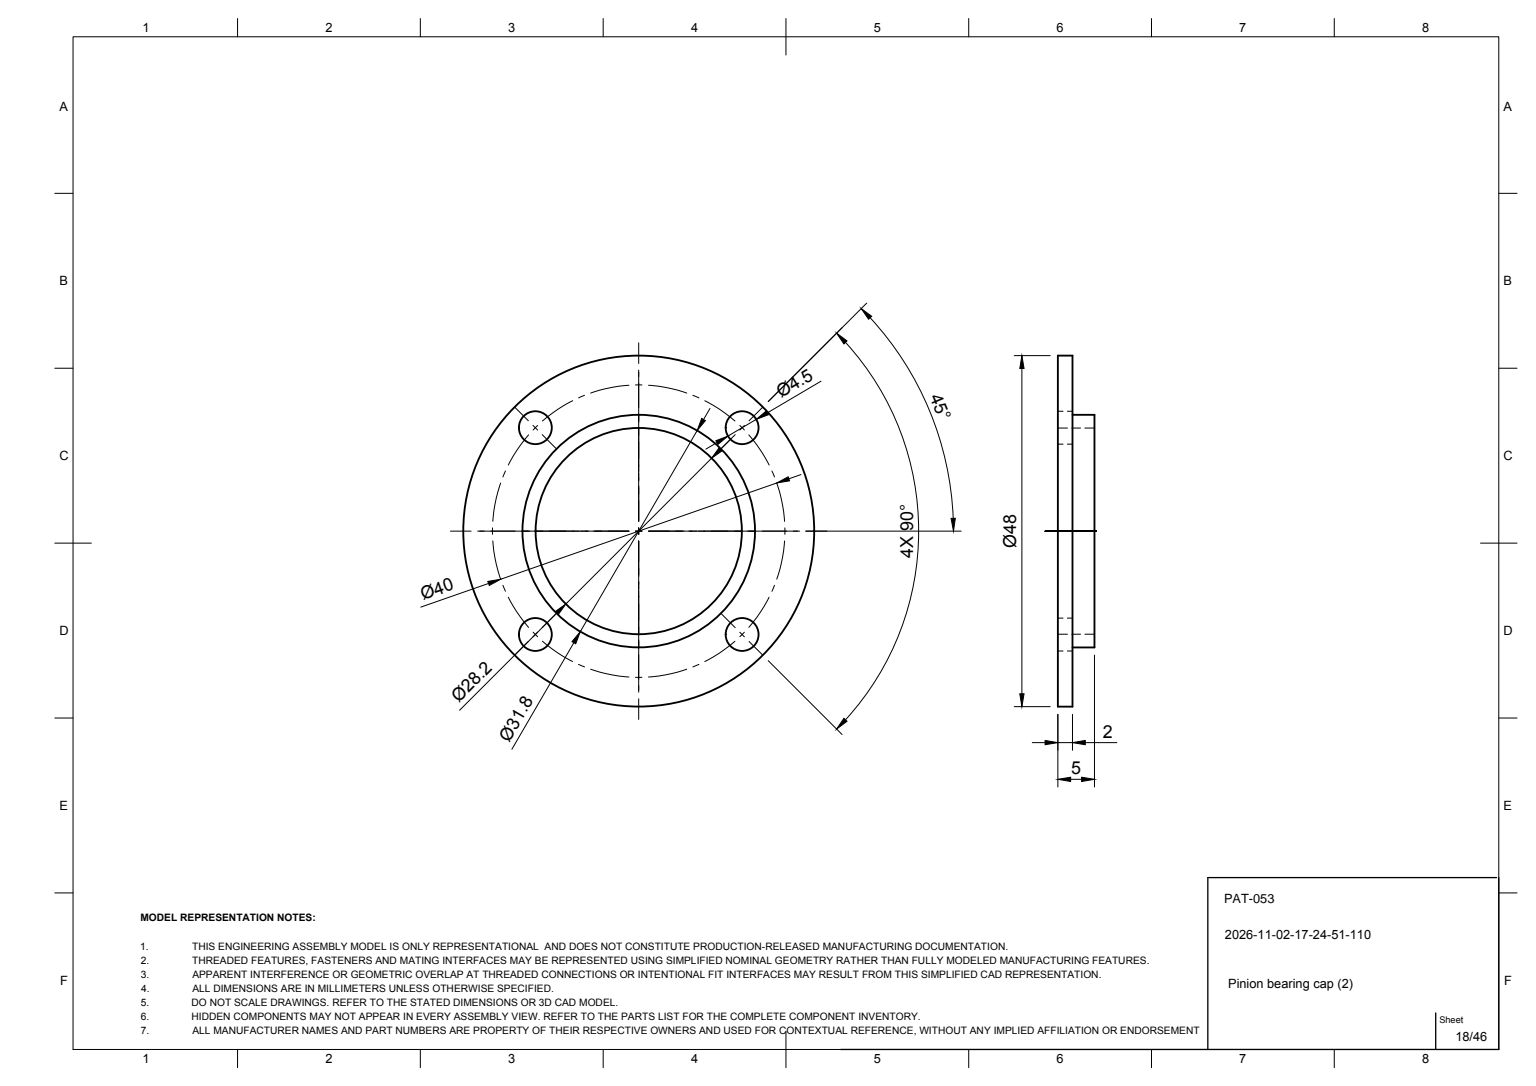
ISO-10303-21;
HEADER;
/* Generated by software containing ST-Developer
 * from STEP Tools, Inc. (www.steptools.com) 
 */

FILE_DESCRIPTION(
/* description */ ('Hand-operated arbor press'),
/* implementation_level */ '2;1');

FILE_NAME(
/* name */ 'Pinion bearing cap (2).step',
/* time_stamp */ '2026-10-28T03:25:25-07:00',
/* author */ (''),
/* organization */ (''),
/* preprocessor_version */ 'ST-DEVELOPER v20.2',
/* originating_system */ 'Autodesk Translation Framework v15.17.0.0',
/* authorisation */ '');

FILE_SCHEMA (('AUTOMOTIVE_DESIGN { 1 0 10303 214 3 1 1 }'));
ENDSEC;

DATA;
#10=MECHANICAL_DESIGN_GEOMETRIC_PRESENTATION_REPRESENTATION('',(#599),#32751);
#515=SHAPE_REPRESENTATION_RELATIONSHIP('SRR','None',#32944,#557);
#557=ADVANCED_BREP_SHAPE_REPRESENTATION('',(#648),#32718);
#599=STYLED_ITEM('',(#33242),#648);
#648=MANIFOLD_SOLID_BREP('Body1',#12496);
#779=FACE_BOUND('',#2262,.T.);
#780=FACE_BOUND('',#2265,.T.);
#781=FACE_BOUND('',#2266,.T.);
#782=FACE_BOUND('',#2267,.T.);
#783=FACE_BOUND('',#2268,.T.);
#784=FACE_BOUND('',#2269,.T.);
#785=FACE_BOUND('',#2271,.T.);
#786=FACE_BOUND('',#2272,.T.);
#787=FACE_BOUND('',#2273,.T.);
#788=FACE_BOUND('',#2274,.T.);
#789=FACE_BOUND('',#2275,.T.);
#960=PLANE('',#13357);
#961=PLANE('',#13361);
#962=PLANE('',#13362);
#1475=FACE_OUTER_BOUND('',#2255,.T.);
#1476=FACE_OUTER_BOUND('',#2256,.T.);
#1477=FACE_OUTER_BOUND('',#2257,.T.);
#1478=FACE_OUTER_BOUND('',#2258,.T.);
#1479=FACE_OUTER_BOUND('',#2259,.T.);
#1480=FACE_OUTER_BOUND('',#2260,.T.);
#1481=FACE_OUTER_BOUND('',#2261,.T.);
#1482=FACE_OUTER_BOUND('',#2263,.T.);
#1483=FACE_OUTER_BOUND('',#2264,.T.);
#1484=FACE_OUTER_BOUND('',#2270,.T.);
#2255=EDGE_LOOP('',(#9194,#9195,#9196,#9197));
#2256=EDGE_LOOP('',(#9198,#9199,#9200,#9201));
#2257=EDGE_LOOP('',(#9202,#9203,#9204,#9205));
#2258=EDGE_LOOP('',(#9206,#9207,#9208,#9209));
#2259=EDGE_LOOP('',(#9210,#9211,#9212,#9213));
#2260=EDGE_LOOP('',(#9214,#9215,#9216,#9217));
#2261=EDGE_LOOP('',(#9218));
#2262=EDGE_LOOP('',(#9219));
#2263=EDGE_LOOP('',(#9220,#9221,#9222,#9223));
#2264=EDGE_LOOP('',(#9224));
#2265=EDGE_LOOP('',(#9225));
#2266=EDGE_LOOP('',(#9226));
#2267=EDGE_LOOP('',(#9227));
#2268=EDGE_LOOP('',(#9228));
#2269=EDGE_LOOP('',(#9229));
#2270=EDGE_LOOP('',(#9230));
#2271=EDGE_LOOP('',(#9231));
#2272=EDGE_LOOP('',(#9232));
#2273=EDGE_LOOP('',(#9233));
#2274=EDGE_LOOP('',(#9234));
#2275=EDGE_LOOP('',(#9235));
#3117=LINE('',#18565,#4288);
#3118=LINE('',#18571,#4289);
#3119=LINE('',#18577,#4290);
#3120=LINE('',#18583,#4291);
#3121=LINE('',#18589,#4292);
#3122=LINE('',#18595,#4293);
#3123=LINE('',#18602,#4294);
#4288=VECTOR('',#15132,1.41);
#4289=VECTOR('',#15139,0.225);
#4290=VECTOR('',#15146,0.225);
#4291=VECTOR('',#15153,0.225);
#4292=VECTOR('',#15160,0.225);
#4293=VECTOR('',#15167,1.59);
#4294=VECTOR('',#15176,2.4);
#5308=CIRCLE('',#13340,1.41);
#5309=CIRCLE('',#13341,1.41);
#5310=CIRCLE('',#13343,0.225);
#5311=CIRCLE('',#13344,0.225);
#5312=CIRCLE('',#13346,0.225);
#5313=CIRCLE('',#13347,0.225);
#5314=CIRCLE('',#13349,0.225);
#5315=CIRCLE('',#13350,0.225);
#5316=CIRCLE('',#13352,0.225);
#5317=CIRCLE('',#13353,0.225);
#5318=CIRCLE('',#13355,1.59);
#5319=CIRCLE('',#13356,1.59);
#5320=CIRCLE('',#13359,2.4);
#5321=CIRCLE('',#13360,2.4);
#5846=VERTEX_POINT('',#18562);
#5847=VERTEX_POINT('',#18564);
#5848=VERTEX_POINT('',#18568);
#5849=VERTEX_POINT('',#18570);
#5850=VERTEX_POINT('',#18574);
#5851=VERTEX_POINT('',#18576);
#5852=VERTEX_POINT('',#18580);
#5853=VERTEX_POINT('',#18582);
#5854=VERTEX_POINT('',#18586);
#5855=VERTEX_POINT('',#18588);
#5856=VERTEX_POINT('',#18592);
#5857=VERTEX_POINT('',#18594);
#5858=VERTEX_POINT('',#18599);
#5859=VERTEX_POINT('',#18601);
#7100=EDGE_CURVE('',#5846,#5846,#5308,.T.);
#7101=EDGE_CURVE('',#5846,#5847,#3117,.T.);
#7102=EDGE_CURVE('',#5847,#5847,#5309,.T.);
#7103=EDGE_CURVE('',#5848,#5848,#5310,.T.);
#7104=EDGE_CURVE('',#5848,#5849,#3118,.T.);
#7105=EDGE_CURVE('',#5849,#5849,#5311,.T.);
#7106=EDGE_CURVE('',#5850,#5850,#5312,.T.);
#7107=EDGE_CURVE('',#5850,#5851,#3119,.T.);
#7108=EDGE_CURVE('',#5851,#5851,#5313,.T.);
#7109=EDGE_CURVE('',#5852,#5852,#5314,.T.);
#7110=EDGE_CURVE('',#5852,#5853,#3120,.T.);
#7111=EDGE_CURVE('',#5853,#5853,#5315,.T.);
#7112=EDGE_CURVE('',#5854,#5854,#5316,.T.);
#7113=EDGE_CURVE('',#5854,#5855,#3121,.T.);
#7114=EDGE_CURVE('',#5855,#5855,#5317,.T.);
#7115=EDGE_CURVE('',#5856,#5856,#5318,.T.);
#7116=EDGE_CURVE('',#5856,#5857,#3122,.T.);
#7117=EDGE_CURVE('',#5857,#5857,#5319,.T.);
#7118=EDGE_CURVE('',#5858,#5858,#5320,.T.);
#7119=EDGE_CURVE('',#5858,#5859,#3123,.T.);
#7120=EDGE_CURVE('',#5859,#5859,#5321,.T.);
#9194=ORIENTED_EDGE('',*,*,#7100,.F.);
#9195=ORIENTED_EDGE('',*,*,#7101,.T.);
#9196=ORIENTED_EDGE('',*,*,#7102,.F.);
#9197=ORIENTED_EDGE('',*,*,#7101,.F.);
#9198=ORIENTED_EDGE('',*,*,#7103,.F.);
#9199=ORIENTED_EDGE('',*,*,#7104,.T.);
#9200=ORIENTED_EDGE('',*,*,#7105,.F.);
#9201=ORIENTED_EDGE('',*,*,#7104,.F.);
#9202=ORIENTED_EDGE('',*,*,#7106,.F.);
#9203=ORIENTED_EDGE('',*,*,#7107,.T.);
#9204=ORIENTED_EDGE('',*,*,#7108,.F.);
#9205=ORIENTED_EDGE('',*,*,#7107,.F.);
#9206=ORIENTED_EDGE('',*,*,#7109,.F.);
#9207=ORIENTED_EDGE('',*,*,#7110,.T.);
#9208=ORIENTED_EDGE('',*,*,#7111,.F.);
#9209=ORIENTED_EDGE('',*,*,#7110,.F.);
#9210=ORIENTED_EDGE('',*,*,#7112,.F.);
#9211=ORIENTED_EDGE('',*,*,#7113,.T.);
#9212=ORIENTED_EDGE('',*,*,#7114,.F.);
#9213=ORIENTED_EDGE('',*,*,#7113,.F.);
#9214=ORIENTED_EDGE('',*,*,#7115,.F.);
#9215=ORIENTED_EDGE('',*,*,#7116,.T.);
#9216=ORIENTED_EDGE('',*,*,#7117,.F.);
#9217=ORIENTED_EDGE('',*,*,#7116,.F.);
#9218=ORIENTED_EDGE('',*,*,#7115,.T.);
#9219=ORIENTED_EDGE('',*,*,#7102,.T.);
#9220=ORIENTED_EDGE('',*,*,#7118,.F.);
#9221=ORIENTED_EDGE('',*,*,#7119,.T.);
#9222=ORIENTED_EDGE('',*,*,#7120,.T.);
#9223=ORIENTED_EDGE('',*,*,#7119,.F.);
#9224=ORIENTED_EDGE('',*,*,#7118,.T.);
#9225=ORIENTED_EDGE('',*,*,#7117,.T.);
#9226=ORIENTED_EDGE('',*,*,#7114,.T.);
#9227=ORIENTED_EDGE('',*,*,#7111,.T.);
#9228=ORIENTED_EDGE('',*,*,#7108,.T.);
#9229=ORIENTED_EDGE('',*,*,#7105,.T.);
#9230=ORIENTED_EDGE('',*,*,#7120,.F.);
#9231=ORIENTED_EDGE('',*,*,#7100,.T.);
#9232=ORIENTED_EDGE('',*,*,#7112,.T.);
#9233=ORIENTED_EDGE('',*,*,#7109,.T.);
#9234=ORIENTED_EDGE('',*,*,#7106,.T.);
#9235=ORIENTED_EDGE('',*,*,#7103,.T.);
#11713=CYLINDRICAL_SURFACE('',#13339,1.41);
#11714=CYLINDRICAL_SURFACE('',#13342,0.225);
#11715=CYLINDRICAL_SURFACE('',#13345,0.225);
#11716=CYLINDRICAL_SURFACE('',#13348,0.225);
#11717=CYLINDRICAL_SURFACE('',#13351,0.225);
#11718=CYLINDRICAL_SURFACE('',#13354,1.59);
#11719=CYLINDRICAL_SURFACE('',#13358,2.4);
#11984=ADVANCED_FACE('',(#1475),#11713,.F.);
#11985=ADVANCED_FACE('',(#1476),#11714,.F.);
#11986=ADVANCED_FACE('',(#1477),#11715,.F.);
#11987=ADVANCED_FACE('',(#1478),#11716,.F.);
#11988=ADVANCED_FACE('',(#1479),#11717,.F.);
#11989=ADVANCED_FACE('',(#1480),#11718,.T.);
#11990=ADVANCED_FACE('',(#1481,#779),#960,.T.);
#11991=ADVANCED_FACE('',(#1482),#11719,.T.);
#11992=ADVANCED_FACE('',(#1483,#780,#781,#782,#783,#784),#961,.T.);
#11993=ADVANCED_FACE('',(#1484,#785,#786,#787,#788,#789),#962,.F.);
#12496=CLOSED_SHELL('',(#11984,#11985,#11986,#11987,#11988,#11989,#11990,
#11991,#11992,#11993));
#13338=AXIS2_PLACEMENT_3D('',#18560,#15126,#15127);
#13339=AXIS2_PLACEMENT_3D('',#18561,#15128,#15129);
#13340=AXIS2_PLACEMENT_3D('',#18563,#15130,#15131);
#13341=AXIS2_PLACEMENT_3D('',#18566,#15133,#15134);
#13342=AXIS2_PLACEMENT_3D('',#18567,#15135,#15136);
#13343=AXIS2_PLACEMENT_3D('',#18569,#15137,#15138);
#13344=AXIS2_PLACEMENT_3D('',#18572,#15140,#15141);
#13345=AXIS2_PLACEMENT_3D('',#18573,#15142,#15143);
#13346=AXIS2_PLACEMENT_3D('',#18575,#15144,#15145);
#13347=AXIS2_PLACEMENT_3D('',#18578,#15147,#15148);
#13348=AXIS2_PLACEMENT_3D('',#18579,#15149,#15150);
#13349=AXIS2_PLACEMENT_3D('',#18581,#15151,#15152);
#13350=AXIS2_PLACEMENT_3D('',#18584,#15154,#15155);
#13351=AXIS2_PLACEMENT_3D('',#18585,#15156,#15157);
#13352=AXIS2_PLACEMENT_3D('',#18587,#15158,#15159);
#13353=AXIS2_PLACEMENT_3D('',#18590,#15161,#15162);
#13354=AXIS2_PLACEMENT_3D('',#18591,#15163,#15164);
#13355=AXIS2_PLACEMENT_3D('',#18593,#15165,#15166);
#13356=AXIS2_PLACEMENT_3D('',#18596,#15168,#15169);
#13357=AXIS2_PLACEMENT_3D('',#18597,#15170,#15171);
#13358=AXIS2_PLACEMENT_3D('',#18598,#15172,#15173);
#13359=AXIS2_PLACEMENT_3D('',#18600,#15174,#15175);
#13360=AXIS2_PLACEMENT_3D('',#18603,#15177,#15178);
#13361=AXIS2_PLACEMENT_3D('',#18604,#15179,#15180);
#13362=AXIS2_PLACEMENT_3D('',#18605,#15181,#15182);
#15126=DIRECTION('axis',(0.,0.,1.));
#15127=DIRECTION('refdir',(1.,0.,0.));
#15128=DIRECTION('center_axis',(0.,1.,0.));
#15129=DIRECTION('ref_axis',(1.,0.,0.));
#15130=DIRECTION('center_axis',(0.,1.,0.));
#15131=DIRECTION('ref_axis',(1.,0.,0.));
#15132=DIRECTION('',(0.,1.,0.));
#15133=DIRECTION('center_axis',(0.,-1.,0.));
#15134=DIRECTION('ref_axis',(1.,0.,0.));
#15135=DIRECTION('center_axis',(0.,1.,0.));
#15136=DIRECTION('ref_axis',(1.,0.,0.));
#15137=DIRECTION('center_axis',(0.,1.,0.));
#15138=DIRECTION('ref_axis',(1.,0.,0.));
#15139=DIRECTION('',(0.,1.,0.));
#15140=DIRECTION('center_axis',(0.,-1.,0.));
#15141=DIRECTION('ref_axis',(1.,0.,0.));
#15142=DIRECTION('center_axis',(0.,1.,0.));
#15143=DIRECTION('ref_axis',(1.,0.,0.));
#15144=DIRECTION('center_axis',(0.,1.,0.));
#15145=DIRECTION('ref_axis',(1.,0.,0.));
#15146=DIRECTION('',(0.,1.,0.));
#15147=DIRECTION('center_axis',(0.,-1.,0.));
#15148=DIRECTION('ref_axis',(1.,0.,0.));
#15149=DIRECTION('center_axis',(0.,1.,0.));
#15150=DIRECTION('ref_axis',(1.,0.,0.));
#15151=DIRECTION('center_axis',(0.,1.,0.));
#15152=DIRECTION('ref_axis',(1.,0.,0.));
#15153=DIRECTION('',(0.,1.,0.));
#15154=DIRECTION('center_axis',(0.,-1.,0.));
#15155=DIRECTION('ref_axis',(1.,0.,0.));
#15156=DIRECTION('center_axis',(0.,1.,0.));
#15157=DIRECTION('ref_axis',(1.,0.,0.));
#15158=DIRECTION('center_axis',(0.,1.,0.));
#15159=DIRECTION('ref_axis',(1.,0.,0.));
#15160=DIRECTION('',(0.,1.,0.));
#15161=DIRECTION('center_axis',(0.,-1.,0.));
#15162=DIRECTION('ref_axis',(1.,0.,0.));
#15163=DIRECTION('center_axis',(0.,1.,0.));
#15164=DIRECTION('ref_axis',(1.,0.,0.));
#15165=DIRECTION('center_axis',(0.,1.,0.));
#15166=DIRECTION('ref_axis',(1.,0.,0.));
#15167=DIRECTION('',(0.,-1.,0.));
#15168=DIRECTION('center_axis',(0.,-1.,0.));
#15169=DIRECTION('ref_axis',(1.,0.,0.));
#15170=DIRECTION('center_axis',(0.,1.,0.));
#15171=DIRECTION('ref_axis',(1.,0.,0.));
#15172=DIRECTION('center_axis',(0.,1.,0.));
#15173=DIRECTION('ref_axis',(1.,0.,0.));
#15174=DIRECTION('center_axis',(0.,1.,0.));
#15175=DIRECTION('ref_axis',(1.,0.,0.));
#15176=DIRECTION('',(0.,-1.,0.));
#15177=DIRECTION('center_axis',(0.,1.,0.));
#15178=DIRECTION('ref_axis',(1.,0.,0.));
#15179=DIRECTION('center_axis',(0.,1.,0.));
#15180=DIRECTION('ref_axis',(1.,0.,0.));
#15181=DIRECTION('center_axis',(0.,1.,0.));
#15182=DIRECTION('ref_axis',(1.,0.,0.));
#18560=CARTESIAN_POINT('',(0.,0.,0.));
#18561=CARTESIAN_POINT('Origin',(-3.25,-4.1,20.));
#18562=CARTESIAN_POINT('',(-4.66,2.,20.));
#18563=CARTESIAN_POINT('Origin',(-3.25,2.,20.));
#18564=CARTESIAN_POINT('',(-4.66,2.5,20.));
#18565=CARTESIAN_POINT('',(-4.66,-4.1,20.));
#18566=CARTESIAN_POINT('Origin',(-3.25,2.5,20.));
#18567=CARTESIAN_POINT('Origin',(-4.66421356237309,1.9,18.5857864376269));
#18568=CARTESIAN_POINT('',(-4.88921356237309,2.,18.5857864376269));
#18569=CARTESIAN_POINT('Origin',(-4.66421356237309,2.,18.5857864376269));
#18570=CARTESIAN_POINT('',(-4.88921356237309,2.2,18.5857864376269));
#18571=CARTESIAN_POINT('',(-4.88921356237309,1.9,18.5857864376269));
#18572=CARTESIAN_POINT('Origin',(-4.66421356237309,2.2,18.5857864376269));
#18573=CARTESIAN_POINT('Origin',(-4.66421356237309,1.9,21.4142135623731));
#18574=CARTESIAN_POINT('',(-4.88921356237309,2.,21.4142135623731));
#18575=CARTESIAN_POINT('Origin',(-4.66421356237309,2.,21.4142135623731));
#18576=CARTESIAN_POINT('',(-4.88921356237309,2.2,21.4142135623731));
#18577=CARTESIAN_POINT('',(-4.88921356237309,1.9,21.4142135623731));
#18578=CARTESIAN_POINT('Origin',(-4.66421356237309,2.2,21.4142135623731));
#18579=CARTESIAN_POINT('Origin',(-1.8357864376269,1.9,21.4142135623731));
#18580=CARTESIAN_POINT('',(-2.0607864376269,2.,21.4142135623731));
#18581=CARTESIAN_POINT('Origin',(-1.8357864376269,2.,21.4142135623731));
#18582=CARTESIAN_POINT('',(-2.0607864376269,2.2,21.4142135623731));
#18583=CARTESIAN_POINT('',(-2.0607864376269,1.9,21.4142135623731));
#18584=CARTESIAN_POINT('Origin',(-1.8357864376269,2.2,21.4142135623731));
#18585=CARTESIAN_POINT('Origin',(-1.83578643762691,1.9,18.5857864376269));
#18586=CARTESIAN_POINT('',(-2.06078643762691,2.,18.5857864376269));
#18587=CARTESIAN_POINT('Origin',(-1.83578643762691,2.,18.5857864376269));
#18588=CARTESIAN_POINT('',(-2.06078643762691,2.2,18.5857864376269));
#18589=CARTESIAN_POINT('',(-2.06078643762691,1.9,18.5857864376269));
#18590=CARTESIAN_POINT('Origin',(-1.83578643762691,2.2,18.5857864376269));
#18591=CARTESIAN_POINT('Origin',(-3.25,2.2,20.));
#18592=CARTESIAN_POINT('',(-4.84,2.5,20.));
#18593=CARTESIAN_POINT('Origin',(-3.25,2.5,20.));
#18594=CARTESIAN_POINT('',(-4.84,2.2,20.));
#18595=CARTESIAN_POINT('',(-4.84,2.2,20.));
#18596=CARTESIAN_POINT('Origin',(-3.25,2.2,20.));
#18597=CARTESIAN_POINT('Origin',(-3.25,2.5,20.));
#18598=CARTESIAN_POINT('Origin',(-3.25,2.,20.));
#18599=CARTESIAN_POINT('',(-5.65,2.2,20.));
#18600=CARTESIAN_POINT('Origin',(-3.25,2.2,20.));
#18601=CARTESIAN_POINT('',(-5.65,2.,20.));
#18602=CARTESIAN_POINT('',(-5.65,2.,20.));
#18603=CARTESIAN_POINT('Origin',(-3.25,2.,20.));
#18604=CARTESIAN_POINT('Origin',(-3.25,2.2,20.));
#18605=CARTESIAN_POINT('Origin',(-3.25,2.,20.));
#32669=UNCERTAINTY_MEASURE_WITH_UNIT(LENGTH_MEASURE(0.001),#32752,
'DISTANCE_ACCURACY_VALUE',
'Maximum model space distance between geometric entities at asserted c
onnectivities');
#32702=UNCERTAINTY_MEASURE_WITH_UNIT(LENGTH_MEASURE(0.001),#32752,
'DISTANCE_ACCURACY_VALUE',
'Maximum model space distance between geometric entities at asserted c
onnectivities');
#32718=(
GEOMETRIC_REPRESENTATION_CONTEXT(3)
GLOBAL_UNCERTAINTY_ASSIGNED_CONTEXT((#32669))
GLOBAL_UNIT_ASSIGNED_CONTEXT((#32752,#32754,#32755))
REPRESENTATION_CONTEXT('','3D')
);
#32751=(
GEOMETRIC_REPRESENTATION_CONTEXT(3)
GLOBAL_UNCERTAINTY_ASSIGNED_CONTEXT((#32702))
GLOBAL_UNIT_ASSIGNED_CONTEXT((#32752,#32754,#32755))
REPRESENTATION_CONTEXT('','3D')
);
#32752=(
LENGTH_UNIT()
NAMED_UNIT(*)
SI_UNIT(.CENTI.,.METRE.)
);
#32754=(
NAMED_UNIT(*)
PLANE_ANGLE_UNIT()
SI_UNIT($,.RADIAN.)
);
#32755=(
NAMED_UNIT(*)
SI_UNIT($,.STERADIAN.)
SOLID_ANGLE_UNIT()
);
#32771=SHAPE_DEFINITION_REPRESENTATION(#32819,#32944);
#32819=PRODUCT_DEFINITION_SHAPE('',$,#32993);
#32944=SHAPE_REPRESENTATION('',(#13338),#32718);
#32977=PRODUCT_DEFINITION_CONTEXT('part definition',#33123,'design');
#32993=PRODUCT_DEFINITION('Pinion bearing cap (2)',
'Pinion bearing cap (2)',#33041,#32977);
#33041=PRODUCT_DEFINITION_FORMATION('',$,#33140);
#33123=APPLICATION_CONTEXT(
'Core Data for Automotive Mechanical Design Process');
#33124=PRODUCT_CONTEXT('part definition',#33123,'mechanical');
#33140=PRODUCT('Pinion bearing cap (2)','Pinion bearing cap (2)',
'Pinion bearing cap (2)',(#33124));
#33236=COLOUR_RGB('Grey',0.48,0.52,0.57);
#33237=FILL_AREA_STYLE_COLOUR('',#33236);
#33238=FILL_AREA_STYLE('',(#33237));
#33239=SURFACE_STYLE_FILL_AREA(#33238);
#33240=SURFACE_SIDE_STYLE('',(#33239));
#33241=SURFACE_STYLE_USAGE(.BOTH.,#33240);
#33242=PRESENTATION_STYLE_ASSIGNMENT((#33241));
ENDSEC;
END-ISO-10303-21;
